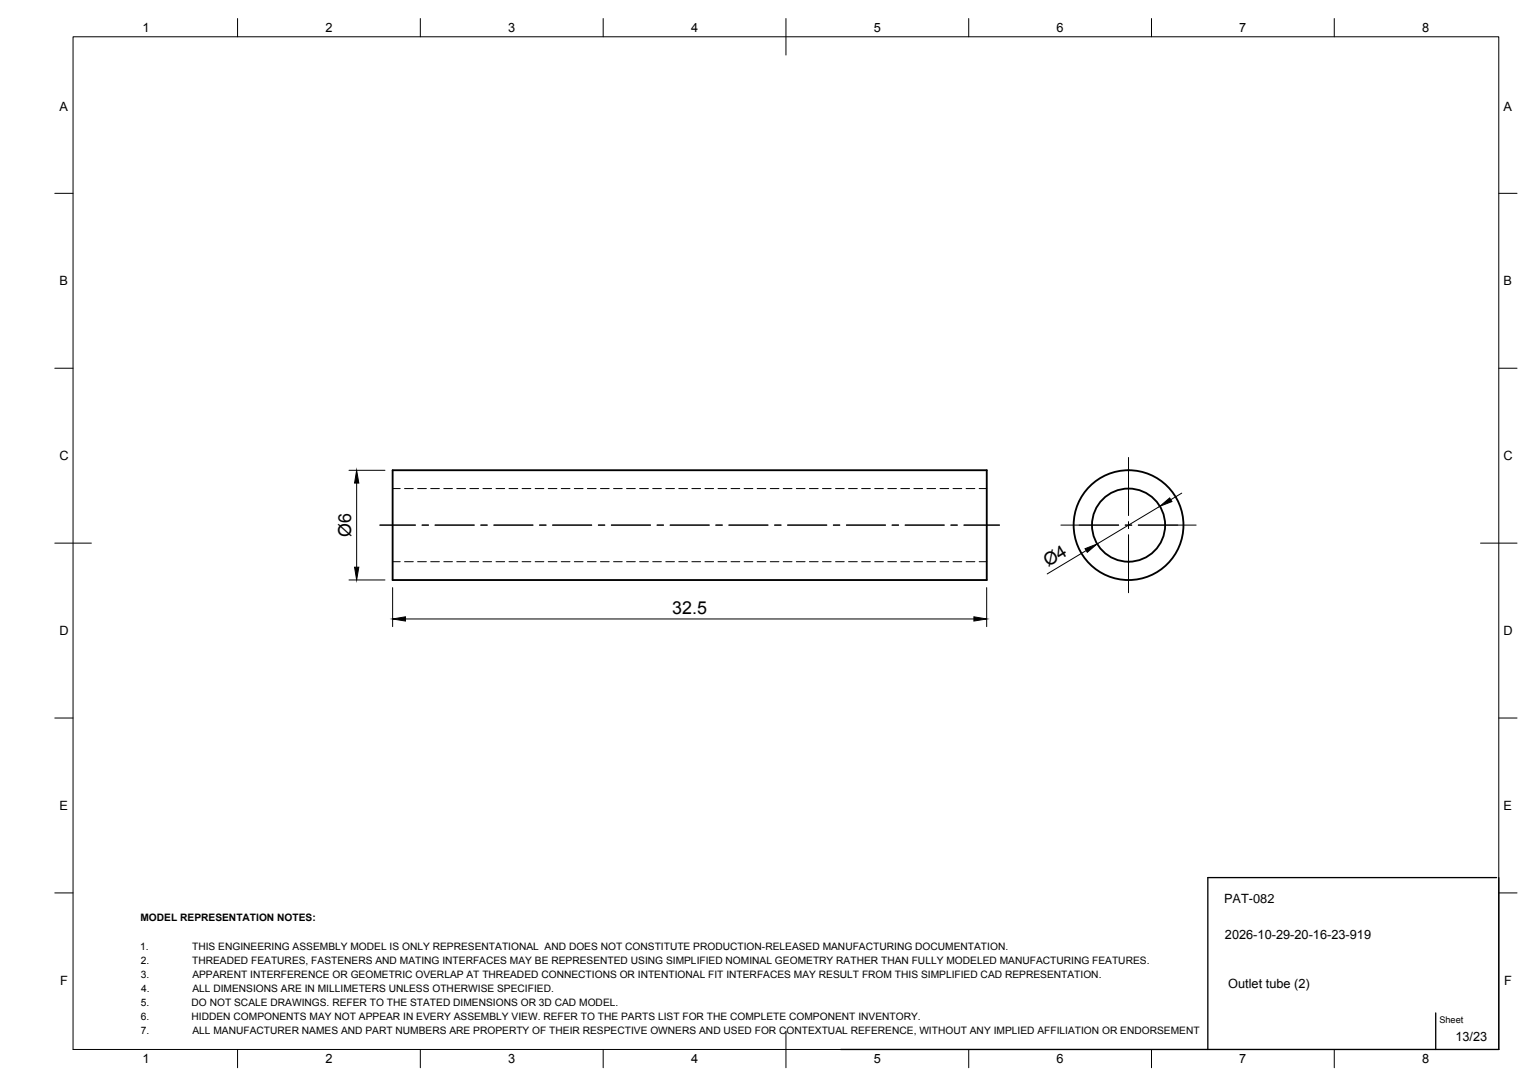
ISO-10303-21;
HEADER;
/* Generated by software containing ST-Developer
 * from STEP Tools, Inc. (www.steptools.com) 
 */

FILE_DESCRIPTION(
/* description */ ('PAT-082'),
/* implementation_level */ '2;1');

FILE_NAME(
/* name */ 'Outlet tube (2).step',
/* time_stamp */ '2026-10-29T20:16:13-07:00',
/* author */ (''),
/* organization */ (''),
/* preprocessor_version */ 'ST-DEVELOPER v20.2',
/* originating_system */ 'Autodesk Translation Framework v15.17.0.0',
/* authorisation */ '');

FILE_SCHEMA (('AUTOMOTIVE_DESIGN { 1 0 10303 214 3 1 1 }'));
ENDSEC;

DATA;
#10=MECHANICAL_DESIGN_GEOMETRIC_PRESENTATION_REPRESENTATION('',(#251),#8266);
#207=SHAPE_REPRESENTATION_RELATIONSHIP('SRR','None',#8369,#229);
#229=ADVANCED_BREP_SHAPE_REPRESENTATION('',(#273),#8253);
#251=STYLED_ITEM('',(#8530),#273);
#273=MANIFOLD_SOLID_BREP('Body1',#4591);
#380=FACE_BOUND('',#1094,.T.);
#381=FACE_BOUND('',#1096,.T.);
#491=PLANE('',#5154);
#492=PLANE('',#5155);
#723=FACE_OUTER_BOUND('',#1091,.T.);
#724=FACE_OUTER_BOUND('',#1092,.T.);
#725=FACE_OUTER_BOUND('',#1093,.T.);
#726=FACE_OUTER_BOUND('',#1095,.T.);
#1091=EDGE_LOOP('',(#3776,#3777,#3778,#3779));
#1092=EDGE_LOOP('',(#3780,#3781,#3782,#3783));
#1093=EDGE_LOOP('',(#3784));
#1094=EDGE_LOOP('',(#3785));
#1095=EDGE_LOOP('',(#3786));
#1096=EDGE_LOOP('',(#3787));
#1432=LINE('',#7685,#1787);
#1433=LINE('',#7691,#1788);
#1787=VECTOR('',#6181,0.2);
#1788=VECTOR('',#6188,0.3);
#2081=CIRCLE('',#5149,0.2);
#2082=CIRCLE('',#5150,0.2);
#2083=CIRCLE('',#5152,0.3);
#2084=CIRCLE('',#5153,0.3);
#2375=VERTEX_POINT('',#7682);
#2376=VERTEX_POINT('',#7684);
#2377=VERTEX_POINT('',#7688);
#2378=VERTEX_POINT('',#7690);
#2864=EDGE_CURVE('',#2375,#2375,#2081,.T.);
#2865=EDGE_CURVE('',#2375,#2376,#1432,.T.);
#2866=EDGE_CURVE('',#2376,#2376,#2082,.T.);
#2867=EDGE_CURVE('',#2377,#2377,#2083,.T.);
#2868=EDGE_CURVE('',#2377,#2378,#1433,.T.);
#2869=EDGE_CURVE('',#2378,#2378,#2084,.T.);
#3776=ORIENTED_EDGE('',*,*,#2864,.F.);
#3777=ORIENTED_EDGE('',*,*,#2865,.T.);
#3778=ORIENTED_EDGE('',*,*,#2866,.T.);
#3779=ORIENTED_EDGE('',*,*,#2865,.F.);
#3780=ORIENTED_EDGE('',*,*,#2867,.F.);
#3781=ORIENTED_EDGE('',*,*,#2868,.T.);
#3782=ORIENTED_EDGE('',*,*,#2869,.T.);
#3783=ORIENTED_EDGE('',*,*,#2868,.F.);
#3784=ORIENTED_EDGE('',*,*,#2867,.T.);
#3785=ORIENTED_EDGE('',*,*,#2864,.T.);
#3786=ORIENTED_EDGE('',*,*,#2869,.F.);
#3787=ORIENTED_EDGE('',*,*,#2866,.F.);
#4285=CYLINDRICAL_SURFACE('',#5148,0.2);
#4286=CYLINDRICAL_SURFACE('',#5151,0.3);
#4462=ADVANCED_FACE('',(#723),#4285,.F.);
#4463=ADVANCED_FACE('',(#724),#4286,.T.);
#4464=ADVANCED_FACE('',(#725,#380),#491,.T.);
#4465=ADVANCED_FACE('',(#726,#381),#492,.F.);
#4591=CLOSED_SHELL('',(#4462,#4463,#4464,#4465));
#5147=AXIS2_PLACEMENT_3D('',#7680,#6175,#6176);
#5148=AXIS2_PLACEMENT_3D('',#7681,#6177,#6178);
#5149=AXIS2_PLACEMENT_3D('',#7683,#6179,#6180);
#5150=AXIS2_PLACEMENT_3D('',#7686,#6182,#6183);
#5151=AXIS2_PLACEMENT_3D('',#7687,#6184,#6185);
#5152=AXIS2_PLACEMENT_3D('',#7689,#6186,#6187);
#5153=AXIS2_PLACEMENT_3D('',#7692,#6189,#6190);
#5154=AXIS2_PLACEMENT_3D('',#7693,#6191,#6192);
#5155=AXIS2_PLACEMENT_3D('',#7694,#6193,#6194);
#6175=DIRECTION('axis',(0.,0.,1.));
#6176=DIRECTION('refdir',(1.,0.,0.));
#6177=DIRECTION('center_axis',(0.,0.,1.));
#6178=DIRECTION('ref_axis',(1.,0.,0.));
#6179=DIRECTION('center_axis',(0.,0.,-1.));
#6180=DIRECTION('ref_axis',(1.,0.,0.));
#6181=DIRECTION('',(0.,0.,-1.));
#6182=DIRECTION('center_axis',(0.,0.,-1.));
#6183=DIRECTION('ref_axis',(1.,0.,0.));
#6184=DIRECTION('center_axis',(0.,0.,1.));
#6185=DIRECTION('ref_axis',(1.,0.,0.));
#6186=DIRECTION('center_axis',(0.,0.,1.));
#6187=DIRECTION('ref_axis',(1.,0.,0.));
#6188=DIRECTION('',(0.,0.,-1.));
#6189=DIRECTION('center_axis',(0.,0.,1.));
#6190=DIRECTION('ref_axis',(1.,0.,0.));
#6191=DIRECTION('center_axis',(0.,0.,1.));
#6192=DIRECTION('ref_axis',(1.,0.,0.));
#6193=DIRECTION('center_axis',(0.,0.,1.));
#6194=DIRECTION('ref_axis',(1.,0.,0.));
#7680=CARTESIAN_POINT('',(0.,0.,0.));
#7681=CARTESIAN_POINT('Origin',(1.25,0.,5.7));
#7682=CARTESIAN_POINT('',(1.05,-2.44929359829471E-17,8.95));
#7683=CARTESIAN_POINT('Origin',(1.25,0.,8.95));
#7684=CARTESIAN_POINT('',(1.05,-2.44929359829471E-17,5.7));
#7685=CARTESIAN_POINT('',(1.05,-2.44929359829471E-17,5.7));
#7686=CARTESIAN_POINT('Origin',(1.25,0.,5.7));
#7687=CARTESIAN_POINT('Origin',(1.25,0.,5.7));
#7688=CARTESIAN_POINT('',(0.95,-3.67394039744206E-17,8.95));
#7689=CARTESIAN_POINT('Origin',(1.25,0.,8.95));
#7690=CARTESIAN_POINT('',(0.95,-3.67394039744206E-17,5.7));
#7691=CARTESIAN_POINT('',(0.95,-3.67394039744206E-17,5.7));
#7692=CARTESIAN_POINT('Origin',(1.25,0.,5.7));
#7693=CARTESIAN_POINT('Origin',(1.25,0.,8.95));
#7694=CARTESIAN_POINT('Origin',(1.25,0.,5.7));
#8228=UNCERTAINTY_MEASURE_WITH_UNIT(LENGTH_MEASURE(0.001),#8267,
'DISTANCE_ACCURACY_VALUE',
'Maximum model space distance between geometric entities at asserted c
onnectivities');
#8241=UNCERTAINTY_MEASURE_WITH_UNIT(LENGTH_MEASURE(0.001),#8267,
'DISTANCE_ACCURACY_VALUE',
'Maximum model space distance between geometric entities at asserted c
onnectivities');
#8253=(
GEOMETRIC_REPRESENTATION_CONTEXT(3)
GLOBAL_UNCERTAINTY_ASSIGNED_CONTEXT((#8228))
GLOBAL_UNIT_ASSIGNED_CONTEXT((#8267,#8269,#8270))
REPRESENTATION_CONTEXT('','3D')
);
#8266=(
GEOMETRIC_REPRESENTATION_CONTEXT(3)
GLOBAL_UNCERTAINTY_ASSIGNED_CONTEXT((#8241))
GLOBAL_UNIT_ASSIGNED_CONTEXT((#8267,#8269,#8270))
REPRESENTATION_CONTEXT('','3D')
);
#8267=(
LENGTH_UNIT()
NAMED_UNIT(*)
SI_UNIT(.CENTI.,.METRE.)
);
#8269=(
NAMED_UNIT(*)
PLANE_ANGLE_UNIT()
SI_UNIT($,.RADIAN.)
);
#8270=(
NAMED_UNIT(*)
SI_UNIT($,.STERADIAN.)
SOLID_ANGLE_UNIT()
);
#8282=SHAPE_DEFINITION_REPRESENTATION(#8306,#8369);
#8306=PRODUCT_DEFINITION_SHAPE('',$,#8394);
#8369=SHAPE_REPRESENTATION('',(#5147),#8253);
#8382=PRODUCT_DEFINITION_CONTEXT('part definition',#8456,'design');
#8394=PRODUCT_DEFINITION('Outlet tube (2)','Outlet tube (2)',
#8418,#8382);
#8418=PRODUCT_DEFINITION_FORMATION('',$,#8469);
#8456=APPLICATION_CONTEXT(
'Core Data for Automotive Mechanical Design Process');
#8457=PRODUCT_CONTEXT('part definition',#8456,'mechanical');
#8469=PRODUCT('Outlet tube (2)','Outlet tube (2)',
'Outlet tube (2)',(#8457));
#8524=COLOUR_RGB('Sky Blue',0.24,0.69,0.87);
#8525=FILL_AREA_STYLE_COLOUR('',#8524);
#8526=FILL_AREA_STYLE('',(#8525));
#8527=SURFACE_STYLE_FILL_AREA(#8526);
#8528=SURFACE_SIDE_STYLE('',(#8527));
#8529=SURFACE_STYLE_USAGE(.BOTH.,#8528);
#8530=PRESENTATION_STYLE_ASSIGNMENT((#8529));
ENDSEC;
END-ISO-10303-21;
